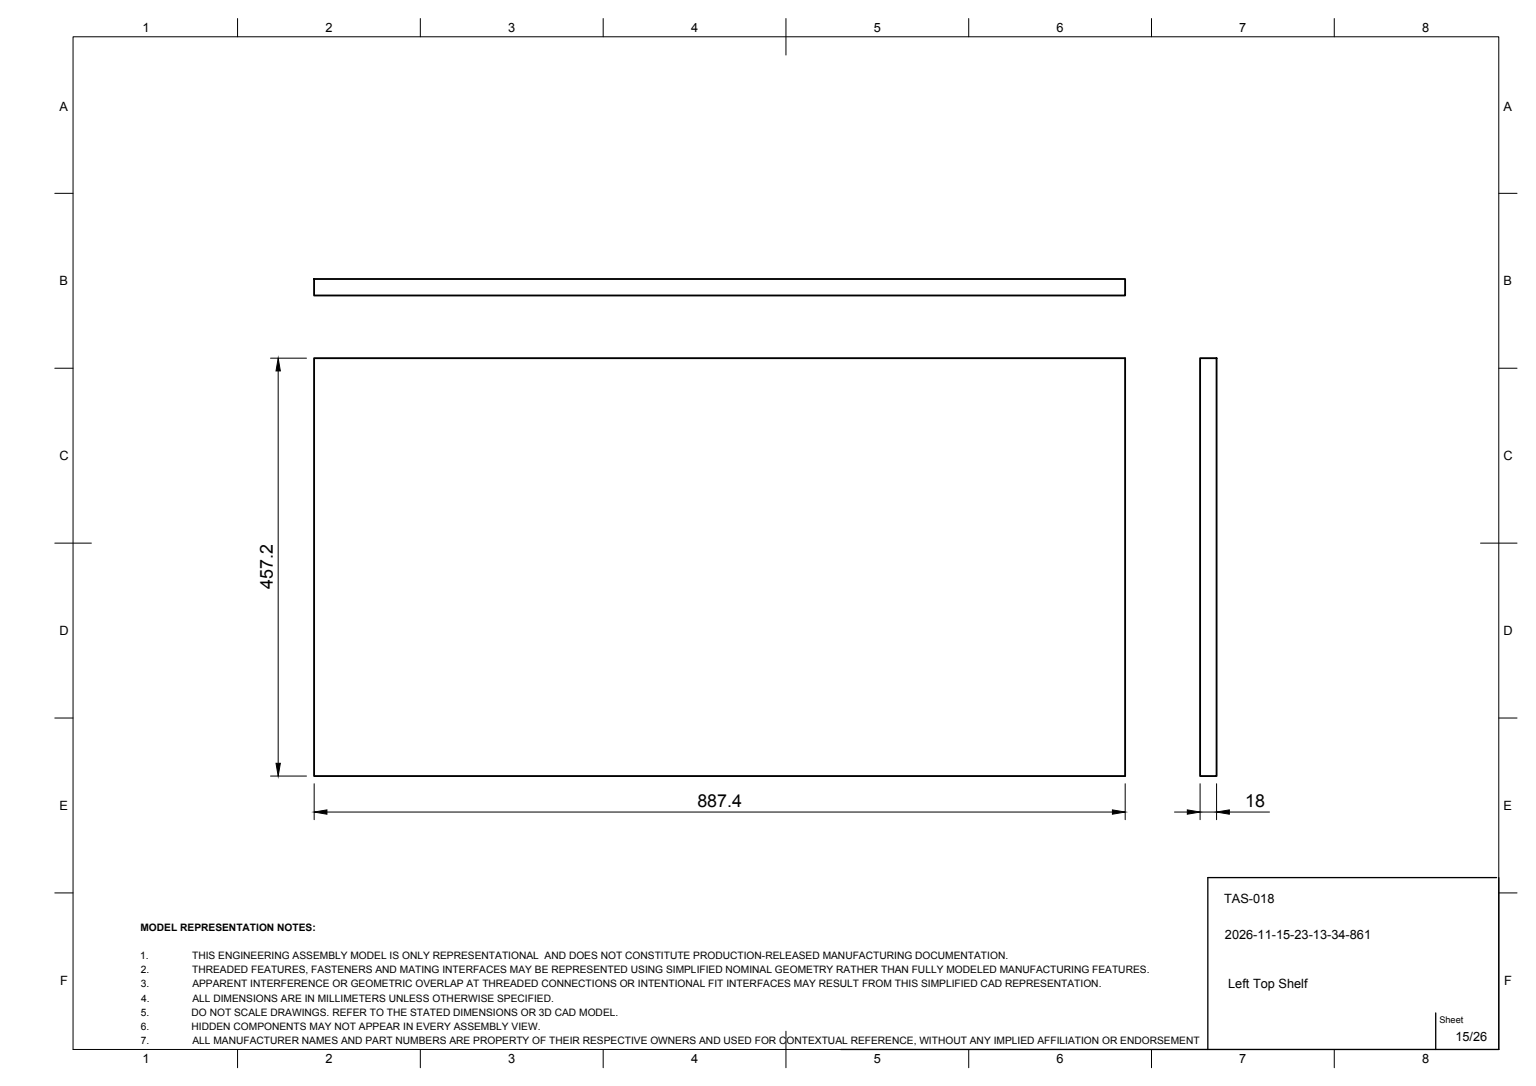
ISO-10303-21;
HEADER;
/* Generated by software containing ST-Developer
 * from STEP Tools, Inc. (www.steptools.com) 
 */

FILE_DESCRIPTION(
/* description */ (''),
/* implementation_level */ '2;1');

FILE_NAME(
/* name */ 'Left Top Shelf.step',
/* time_stamp */ '2026-11-15T15:17:57-08:00',
/* author */ (''),
/* organization */ (''),
/* preprocessor_version */ 'ST-DEVELOPER v20.2',
/* originating_system */ 'Autodesk Translation Framework v15.17.0.0',
/* authorisation */ '');

FILE_SCHEMA (('AUTOMOTIVE_DESIGN { 1 0 10303 214 3 1 1 }'));
ENDSEC;

DATA;
#10=MECHANICAL_DESIGN_GEOMETRIC_PRESENTATION_REPRESENTATION('',(#190),#3723);
#142=SHAPE_REPRESENTATION_RELATIONSHIP('SRR','None',#3823,#166);
#166=ADVANCED_BREP_SHAPE_REPRESENTATION('',(#214),#3712);
#190=STYLED_ITEM('',(#3947),#214);
#214=MANIFOLD_SOLID_BREP('Body1',#2038);
#297=FACE_OUTER_BOUND('',#423,.T.);
#298=FACE_OUTER_BOUND('',#424,.T.);
#299=FACE_OUTER_BOUND('',#425,.T.);
#300=FACE_OUTER_BOUND('',#426,.T.);
#301=FACE_OUTER_BOUND('',#427,.T.);
#302=FACE_OUTER_BOUND('',#428,.T.);
#423=EDGE_LOOP('',(#1587,#1588,#1589,#1590));
#424=EDGE_LOOP('',(#1591,#1592,#1593,#1594));
#425=EDGE_LOOP('',(#1595,#1596,#1597,#1598));
#426=EDGE_LOOP('',(#1599,#1600,#1601,#1602));
#427=EDGE_LOOP('',(#1603,#1604,#1605,#1606));
#428=EDGE_LOOP('',(#1607,#1608,#1609,#1610));
#611=LINE('',#3425,#833);
#612=LINE('',#3427,#834);
#613=LINE('',#3429,#835);
#614=LINE('',#3430,#836);
#615=LINE('',#3433,#837);
#616=LINE('',#3435,#838);
#617=LINE('',#3436,#839);
#618=LINE('',#3439,#840);
#619=LINE('',#3441,#841);
#620=LINE('',#3442,#842);
#621=LINE('',#3444,#843);
#622=LINE('',#3445,#844);
#833=VECTOR('',#2825,0.708661417322839);
#834=VECTOR('',#2826,18.);
#835=VECTOR('',#2827,0.708661417322839);
#836=VECTOR('',#2828,18.);
#837=VECTOR('',#2831,34.9370078740157);
#838=VECTOR('',#2832,18.);
#839=VECTOR('',#2833,34.9370078740157);
#840=VECTOR('',#2836,0.708661417322839);
#841=VECTOR('',#2837,18.);
#842=VECTOR('',#2838,0.708661417322839);
#843=VECTOR('',#2841,34.9370078740157);
#844=VECTOR('',#2842,34.9370078740157);
#1013=VERTEX_POINT('',#3423);
#1014=VERTEX_POINT('',#3424);
#1015=VERTEX_POINT('',#3426);
#1016=VERTEX_POINT('',#3428);
#1017=VERTEX_POINT('',#3432);
#1018=VERTEX_POINT('',#3434);
#1019=VERTEX_POINT('',#3438);
#1020=VERTEX_POINT('',#3440);
#1215=EDGE_CURVE('',#1013,#1014,#611,.T.);
#1216=EDGE_CURVE('',#1015,#1014,#612,.T.);
#1217=EDGE_CURVE('',#1016,#1015,#613,.T.);
#1218=EDGE_CURVE('',#1016,#1013,#614,.T.);
#1219=EDGE_CURVE('',#1014,#1017,#615,.T.);
#1220=EDGE_CURVE('',#1018,#1017,#616,.T.);
#1221=EDGE_CURVE('',#1015,#1018,#617,.T.);
#1222=EDGE_CURVE('',#1017,#1019,#618,.T.);
#1223=EDGE_CURVE('',#1020,#1019,#619,.T.);
#1224=EDGE_CURVE('',#1018,#1020,#620,.T.);
#1225=EDGE_CURVE('',#1013,#1019,#621,.T.);
#1226=EDGE_CURVE('',#1016,#1020,#622,.T.);
#1587=ORIENTED_EDGE('',*,*,#1215,.T.);
#1588=ORIENTED_EDGE('',*,*,#1216,.F.);
#1589=ORIENTED_EDGE('',*,*,#1217,.F.);
#1590=ORIENTED_EDGE('',*,*,#1218,.T.);
#1591=ORIENTED_EDGE('',*,*,#1219,.T.);
#1592=ORIENTED_EDGE('',*,*,#1220,.F.);
#1593=ORIENTED_EDGE('',*,*,#1221,.F.);
#1594=ORIENTED_EDGE('',*,*,#1216,.T.);
#1595=ORIENTED_EDGE('',*,*,#1222,.T.);
#1596=ORIENTED_EDGE('',*,*,#1223,.F.);
#1597=ORIENTED_EDGE('',*,*,#1224,.F.);
#1598=ORIENTED_EDGE('',*,*,#1220,.T.);
#1599=ORIENTED_EDGE('',*,*,#1225,.F.);
#1600=ORIENTED_EDGE('',*,*,#1218,.F.);
#1601=ORIENTED_EDGE('',*,*,#1226,.T.);
#1602=ORIENTED_EDGE('',*,*,#1223,.T.);
#1603=ORIENTED_EDGE('',*,*,#1217,.T.);
#1604=ORIENTED_EDGE('',*,*,#1221,.T.);
#1605=ORIENTED_EDGE('',*,*,#1224,.T.);
#1606=ORIENTED_EDGE('',*,*,#1226,.F.);
#1607=ORIENTED_EDGE('',*,*,#1215,.F.);
#1608=ORIENTED_EDGE('',*,*,#1225,.T.);
#1609=ORIENTED_EDGE('',*,*,#1222,.F.);
#1610=ORIENTED_EDGE('',*,*,#1219,.F.);
#1849=PLANE('',#2407);
#1850=PLANE('',#2408);
#1851=PLANE('',#2409);
#1852=PLANE('',#2410);
#1853=PLANE('',#2411);
#1854=PLANE('',#2412);
#1971=ADVANCED_FACE('',(#297),#1849,.F.);
#1972=ADVANCED_FACE('',(#298),#1850,.F.);
#1973=ADVANCED_FACE('',(#299),#1851,.F.);
#1974=ADVANCED_FACE('',(#300),#1852,.T.);
#1975=ADVANCED_FACE('',(#301),#1853,.T.);
#1976=ADVANCED_FACE('',(#302),#1854,.F.);
#2038=CLOSED_SHELL('',(#1971,#1972,#1973,#1974,#1975,#1976));
#2406=AXIS2_PLACEMENT_3D('',#3421,#2821,#2822);
#2407=AXIS2_PLACEMENT_3D('',#3422,#2823,#2824);
#2408=AXIS2_PLACEMENT_3D('',#3431,#2829,#2830);
#2409=AXIS2_PLACEMENT_3D('',#3437,#2834,#2835);
#2410=AXIS2_PLACEMENT_3D('',#3443,#2839,#2840);
#2411=AXIS2_PLACEMENT_3D('',#3446,#2843,#2844);
#2412=AXIS2_PLACEMENT_3D('',#3447,#2845,#2846);
#2821=DIRECTION('axis',(0.,0.,1.));
#2822=DIRECTION('refdir',(1.,0.,0.));
#2823=DIRECTION('center_axis',(1.,1.17112133399278E-16,0.));
#2824=DIRECTION('ref_axis',(0.,0.,-1.));
#2825=DIRECTION('',(0.,-1.,0.));
#2826=DIRECTION('',(0.,0.,-1.));
#2827=DIRECTION('',(0.,-1.,0.));
#2828=DIRECTION('',(0.,0.,-1.));
#2829=DIRECTION('center_axis',(0.,1.,0.));
#2830=DIRECTION('ref_axis',(0.,0.,1.));
#2831=DIRECTION('',(1.,0.,0.));
#2832=DIRECTION('',(0.,0.,-1.));
#2833=DIRECTION('',(1.,0.,0.));
#2834=DIRECTION('center_axis',(-1.,-9.88133625556409E-17,0.));
#2835=DIRECTION('ref_axis',(0.,0.,1.));
#2836=DIRECTION('',(-1.23358113847239E-16,1.,0.));
#2837=DIRECTION('',(0.,0.,-1.));
#2838=DIRECTION('',(-1.23358113847239E-16,1.,0.));
#2839=DIRECTION('center_axis',(0.,1.,0.));
#2840=DIRECTION('ref_axis',(0.,0.,1.));
#2841=DIRECTION('',(1.,0.,0.));
#2842=DIRECTION('',(1.,0.,0.));
#2843=DIRECTION('center_axis',(0.,0.,1.));
#2844=DIRECTION('ref_axis',(1.,0.,0.));
#2845=DIRECTION('center_axis',(0.,0.,1.));
#2846=DIRECTION('ref_axis',(1.,0.,0.));
#3421=CARTESIAN_POINT('',(0.,0.,0.));
#3422=CARTESIAN_POINT('Origin',(-35.2913385826772,-4.13304395193358E-15,
18.7086614173228));
#3423=CARTESIAN_POINT('',(-35.2913385826772,67.3543307086614,0.708661417322834));
#3424=CARTESIAN_POINT('',(-35.2913385826772,66.6456692913386,0.708661417322834));
#3425=CARTESIAN_POINT('',(-35.2913385826772,67.3543307086614,0.708661417322834));
#3426=CARTESIAN_POINT('',(-35.2913385826772,66.6456692913386,18.7086614173228));
#3427=CARTESIAN_POINT('',(-35.2913385826772,66.6456692913386,18.7086614173228));
#3428=CARTESIAN_POINT('',(-35.2913385826772,67.3543307086614,18.7086614173228));
#3429=CARTESIAN_POINT('',(-35.2913385826772,67.3543307086614,18.7086614173228));
#3430=CARTESIAN_POINT('',(-35.2913385826772,67.3543307086614,18.7086614173228));
#3431=CARTESIAN_POINT('Origin',(0.,66.6456692913386,18.7086614173228));
#3432=CARTESIAN_POINT('',(-0.354330708661425,66.6456692913386,0.708661417322834));
#3433=CARTESIAN_POINT('',(-35.2913385826772,66.6456692913386,0.708661417322834));
#3434=CARTESIAN_POINT('',(-0.354330708661425,66.6456692913386,18.7086614173228));
#3435=CARTESIAN_POINT('',(-0.354330708661425,66.6456692913386,18.7086614173228));
#3436=CARTESIAN_POINT('',(-35.2913385826772,66.6456692913386,18.7086614173228));
#3437=CARTESIAN_POINT('Origin',(-0.354330708661418,-3.50126087795579E-17,
18.7086614173228));
#3438=CARTESIAN_POINT('',(-0.354330708661425,67.3543307086614,0.708661417322834));
#3439=CARTESIAN_POINT('',(-0.354330708661425,66.6456692913386,0.708661417322834));
#3440=CARTESIAN_POINT('',(-0.354330708661425,67.3543307086614,18.7086614173228));
#3441=CARTESIAN_POINT('',(-0.354330708661425,67.3543307086614,18.7086614173228));
#3442=CARTESIAN_POINT('',(-0.354330708661425,66.6456692913386,18.7086614173228));
#3443=CARTESIAN_POINT('Origin',(0.,67.3543307086614,18.7086614173228));
#3444=CARTESIAN_POINT('',(-35.2913385826772,67.3543307086614,0.708661417322834));
#3445=CARTESIAN_POINT('',(-35.2913385826772,67.3543307086614,18.7086614173228));
#3446=CARTESIAN_POINT('Origin',(0.,0.,18.7086614173228));
#3447=CARTESIAN_POINT('Origin',(0.,0.,0.708661417322834));
#3685=UNCERTAINTY_MEASURE_WITH_UNIT(LENGTH_MEASURE(0.000393700787401575),
#3725,'DISTANCE_ACCURACY_VALUE',
'Maximum model space distance between geometric entities at asserted c
onnectivities');
#3696=UNCERTAINTY_MEASURE_WITH_UNIT(LENGTH_MEASURE(0.000393700787401575),
#3725,'DISTANCE_ACCURACY_VALUE',
'Maximum model space distance between geometric entities at asserted c
onnectivities');
#3712=(
GEOMETRIC_REPRESENTATION_CONTEXT(3)
GLOBAL_UNCERTAINTY_ASSIGNED_CONTEXT((#3685))
GLOBAL_UNIT_ASSIGNED_CONTEXT((#3725,#3729,#3730))
REPRESENTATION_CONTEXT('','3D')
);
#3723=(
GEOMETRIC_REPRESENTATION_CONTEXT(3)
GLOBAL_UNCERTAINTY_ASSIGNED_CONTEXT((#3696))
GLOBAL_UNIT_ASSIGNED_CONTEXT((#3725,#3729,#3730))
REPRESENTATION_CONTEXT('','3D')
);
#3724=DIMENSIONAL_EXPONENTS(1.,0.,0.,0.,0.,0.,0.);
#3725=(
CONVERSION_BASED_UNIT('inch',#3728)
LENGTH_UNIT()
NAMED_UNIT(#3724)
);
#3726=(
LENGTH_UNIT()
NAMED_UNIT(*)
SI_UNIT(.MILLI.,.METRE.)
);
#3728=LENGTH_MEASURE_WITH_UNIT(LENGTH_MEASURE(25.4),#3726);
#3729=(
NAMED_UNIT(*)
PLANE_ANGLE_UNIT()
SI_UNIT($,.RADIAN.)
);
#3730=(
NAMED_UNIT(*)
SI_UNIT($,.STERADIAN.)
SOLID_ANGLE_UNIT()
);
#3746=SHAPE_DEFINITION_REPRESENTATION(#3773,#3823);
#3773=PRODUCT_DEFINITION_SHAPE('',$,#3850);
#3823=SHAPE_REPRESENTATION('',(#2406),#3712);
#3834=PRODUCT_DEFINITION_CONTEXT('part definition',#3914,'design');
#3850=PRODUCT_DEFINITION('2026-11-15-23-13-34-861','Left Top Shelf',#3876,
#3834);
#3876=PRODUCT_DEFINITION_FORMATION('',$,#3931);
#3914=APPLICATION_CONTEXT(
'Core Data for Automotive Mechanical Design Process');
#3915=PRODUCT_CONTEXT('part definition',#3914,'mechanical');
#3931=PRODUCT('2026-11-15-23-13-34-861','Left Top Shelf',$,(#3915));
#3947=PRESENTATION_STYLE_ASSIGNMENT((#3955));
#3955=SURFACE_STYLE_USAGE(.BOTH.,#3963);
#3963=SURFACE_SIDE_STYLE('',(#3971));
#3971=SURFACE_STYLE_FILL_AREA(#3979);
#3979=FILL_AREA_STYLE('Light Blue',(#3987));
#3987=FILL_AREA_STYLE_COLOUR('Light Blue',#3995);
#3995=COLOUR_RGB('Light Blue',0.67843137254902,0.847058823529412,0.901960784313726);
ENDSEC;
END-ISO-10303-21;
